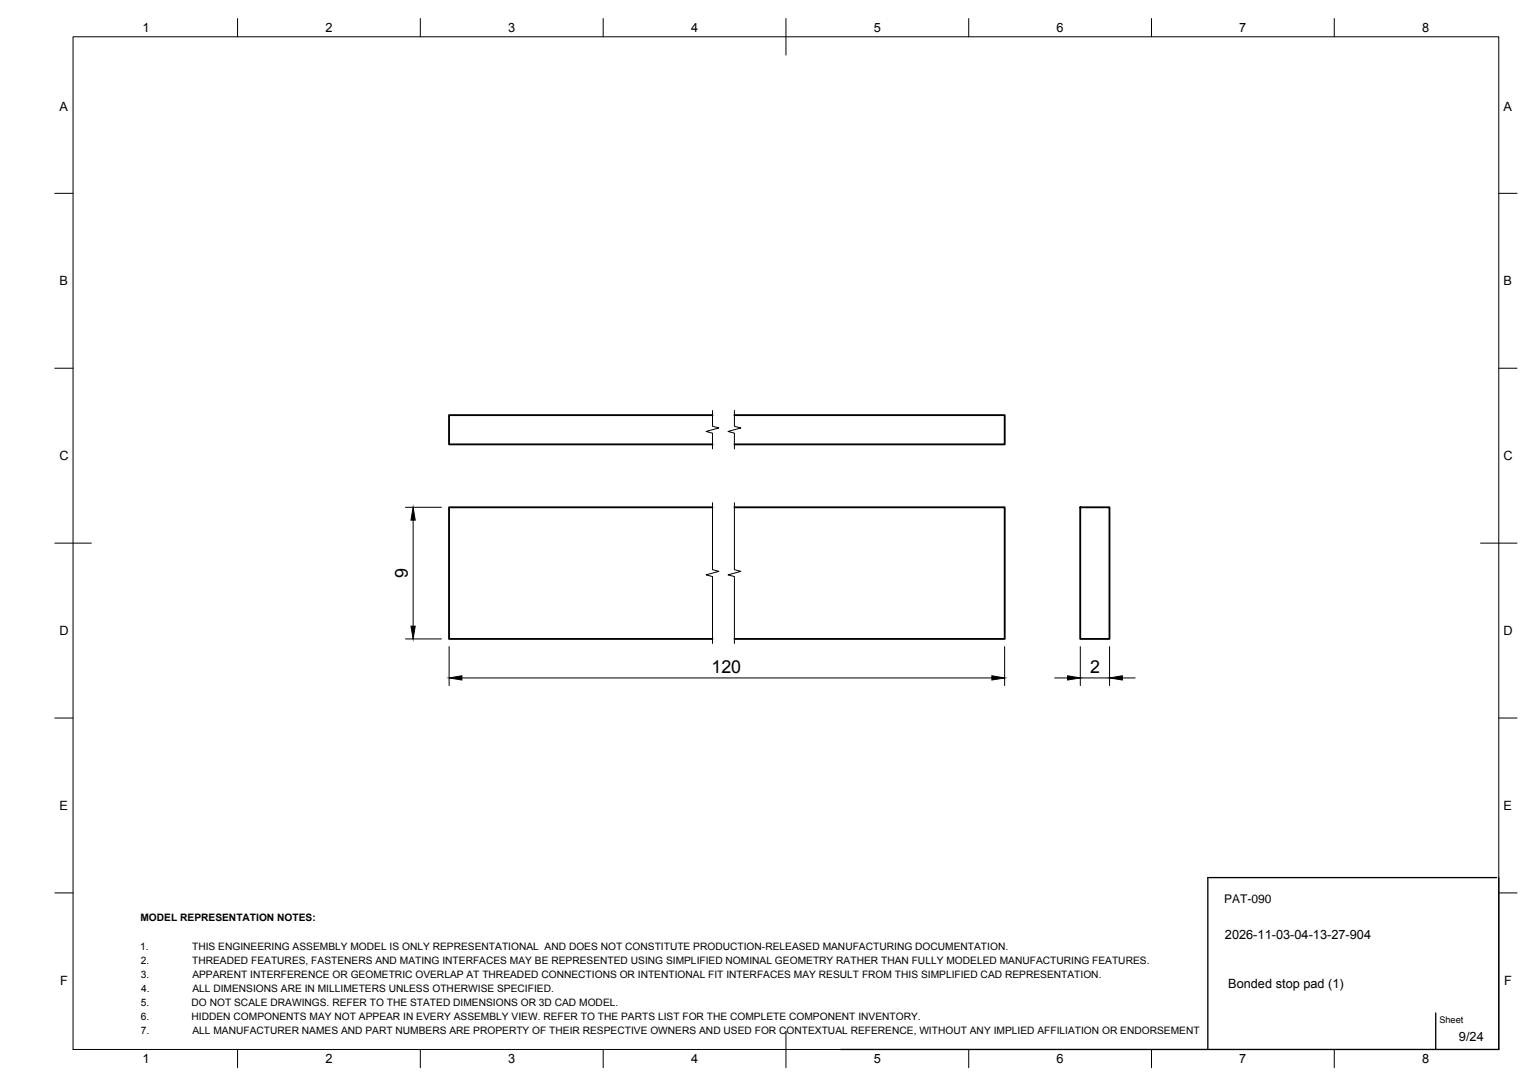
ISO-10303-21;
HEADER;
/* Generated by software containing ST-Developer
 * from STEP Tools, Inc. (www.steptools.com) 
 */

FILE_DESCRIPTION(
/* description */ ('Round-Shaft Linear Stage with Ball Bushings'),
/* implementation_level */ '2;1');

FILE_NAME(
/* name */ 'Bonded stop pad (1).step',
/* time_stamp */ '2026-10-27T10:47:55-07:00',
/* author */ (''),
/* organization */ (''),
/* preprocessor_version */ 'ST-DEVELOPER v20.2',
/* originating_system */ 'Autodesk Translation Framework v15.17.0.0',
/* authorisation */ '');

FILE_SCHEMA (('AUTOMOTIVE_DESIGN { 1 0 10303 214 3 1 1 }'));
ENDSEC;

DATA;
#10=MECHANICAL_DESIGN_GEOMETRIC_PRESENTATION_REPRESENTATION('',(#306),#7835);
#264=SHAPE_REPRESENTATION_RELATIONSHIP('SRR','None',#7952,#285);
#285=ADVANCED_BREP_SHAPE_REPRESENTATION('',(#327),#7816);
#306=STYLED_ITEM('',(#8158),#327);
#327=MANIFOLD_SOLID_BREP('Body1',#4396);
#487=PLANE('',#4744);
#488=PLANE('',#4745);
#489=PLANE('',#4746);
#490=PLANE('',#4747);
#491=PLANE('',#4748);
#492=PLANE('',#4749);
#664=FACE_OUTER_BOUND('',#957,.T.);
#665=FACE_OUTER_BOUND('',#958,.T.);
#666=FACE_OUTER_BOUND('',#959,.T.);
#667=FACE_OUTER_BOUND('',#960,.T.);
#668=FACE_OUTER_BOUND('',#961,.T.);
#669=FACE_OUTER_BOUND('',#962,.T.);
#957=EDGE_LOOP('',(#3210,#3211,#3212,#3213));
#958=EDGE_LOOP('',(#3214,#3215,#3216,#3217));
#959=EDGE_LOOP('',(#3218,#3219,#3220,#3221));
#960=EDGE_LOOP('',(#3222,#3223,#3224,#3225));
#961=EDGE_LOOP('',(#3226,#3227,#3228,#3229));
#962=EDGE_LOOP('',(#3230,#3231,#3232,#3233));
#1317=LINE('',#6808,#1657);
#1318=LINE('',#6810,#1658);
#1319=LINE('',#6812,#1659);
#1320=LINE('',#6813,#1660);
#1321=LINE('',#6816,#1661);
#1322=LINE('',#6818,#1662);
#1323=LINE('',#6819,#1663);
#1324=LINE('',#6822,#1664);
#1325=LINE('',#6824,#1665);
#1326=LINE('',#6825,#1666);
#1327=LINE('',#6827,#1667);
#1328=LINE('',#6828,#1668);
#1657=VECTOR('',#5436,1.);
#1658=VECTOR('',#5437,1.);
#1659=VECTOR('',#5438,1.);
#1660=VECTOR('',#5439,1.);
#1661=VECTOR('',#5442,1.);
#1662=VECTOR('',#5443,1.);
#1663=VECTOR('',#5444,1.);
#1664=VECTOR('',#5447,1.);
#1665=VECTOR('',#5448,1.);
#1666=VECTOR('',#5449,1.);
#1667=VECTOR('',#5452,1.);
#1668=VECTOR('',#5453,1.);
#2190=VERTEX_POINT('',#6806);
#2191=VERTEX_POINT('',#6807);
#2192=VERTEX_POINT('',#6809);
#2193=VERTEX_POINT('',#6811);
#2194=VERTEX_POINT('',#6815);
#2195=VERTEX_POINT('',#6817);
#2196=VERTEX_POINT('',#6821);
#2197=VERTEX_POINT('',#6823);
#2573=EDGE_CURVE('',#2190,#2191,#1317,.T.);
#2574=EDGE_CURVE('',#2191,#2192,#1318,.T.);
#2575=EDGE_CURVE('',#2193,#2192,#1319,.T.);
#2576=EDGE_CURVE('',#2190,#2193,#1320,.T.);
#2577=EDGE_CURVE('',#2194,#2190,#1321,.T.);
#2578=EDGE_CURVE('',#2195,#2193,#1322,.T.);
#2579=EDGE_CURVE('',#2194,#2195,#1323,.T.);
#2580=EDGE_CURVE('',#2196,#2194,#1324,.T.);
#2581=EDGE_CURVE('',#2197,#2195,#1325,.T.);
#2582=EDGE_CURVE('',#2196,#2197,#1326,.T.);
#2583=EDGE_CURVE('',#2191,#2196,#1327,.T.);
#2584=EDGE_CURVE('',#2192,#2197,#1328,.T.);
#3210=ORIENTED_EDGE('',*,*,#2573,.T.);
#3211=ORIENTED_EDGE('',*,*,#2574,.T.);
#3212=ORIENTED_EDGE('',*,*,#2575,.F.);
#3213=ORIENTED_EDGE('',*,*,#2576,.F.);
#3214=ORIENTED_EDGE('',*,*,#2577,.T.);
#3215=ORIENTED_EDGE('',*,*,#2576,.T.);
#3216=ORIENTED_EDGE('',*,*,#2578,.F.);
#3217=ORIENTED_EDGE('',*,*,#2579,.F.);
#3218=ORIENTED_EDGE('',*,*,#2580,.T.);
#3219=ORIENTED_EDGE('',*,*,#2579,.T.);
#3220=ORIENTED_EDGE('',*,*,#2581,.F.);
#3221=ORIENTED_EDGE('',*,*,#2582,.F.);
#3222=ORIENTED_EDGE('',*,*,#2583,.T.);
#3223=ORIENTED_EDGE('',*,*,#2582,.T.);
#3224=ORIENTED_EDGE('',*,*,#2584,.F.);
#3225=ORIENTED_EDGE('',*,*,#2574,.F.);
#3226=ORIENTED_EDGE('',*,*,#2584,.T.);
#3227=ORIENTED_EDGE('',*,*,#2581,.T.);
#3228=ORIENTED_EDGE('',*,*,#2578,.T.);
#3229=ORIENTED_EDGE('',*,*,#2575,.T.);
#3230=ORIENTED_EDGE('',*,*,#2583,.F.);
#3231=ORIENTED_EDGE('',*,*,#2573,.F.);
#3232=ORIENTED_EDGE('',*,*,#2577,.F.);
#3233=ORIENTED_EDGE('',*,*,#2580,.F.);
#4183=ADVANCED_FACE('',(#664),#487,.T.);
#4184=ADVANCED_FACE('',(#665),#488,.T.);
#4185=ADVANCED_FACE('',(#666),#489,.T.);
#4186=ADVANCED_FACE('',(#667),#490,.T.);
#4187=ADVANCED_FACE('',(#668),#491,.T.);
#4188=ADVANCED_FACE('',(#669),#492,.F.);
#4396=CLOSED_SHELL('',(#4183,#4184,#4185,#4186,#4187,#4188));
#4743=AXIS2_PLACEMENT_3D('',#6804,#5432,#5433);
#4744=AXIS2_PLACEMENT_3D('',#6805,#5434,#5435);
#4745=AXIS2_PLACEMENT_3D('',#6814,#5440,#5441);
#4746=AXIS2_PLACEMENT_3D('',#6820,#5445,#5446);
#4747=AXIS2_PLACEMENT_3D('',#6826,#5450,#5451);
#4748=AXIS2_PLACEMENT_3D('',#6829,#5454,#5455);
#4749=AXIS2_PLACEMENT_3D('',#6830,#5456,#5457);
#5432=DIRECTION('axis',(0.,0.,1.));
#5433=DIRECTION('refdir',(1.,0.,0.));
#5434=DIRECTION('center_axis',(0.,1.,0.));
#5435=DIRECTION('ref_axis',(-1.,0.,0.));
#5436=DIRECTION('',(-1.,0.,0.));
#5437=DIRECTION('',(0.,0.,1.));
#5438=DIRECTION('',(-1.,0.,0.));
#5439=DIRECTION('',(0.,0.,1.));
#5440=DIRECTION('center_axis',(1.,0.,0.));
#5441=DIRECTION('ref_axis',(0.,1.,0.));
#5442=DIRECTION('',(0.,1.,0.));
#5443=DIRECTION('',(0.,1.,0.));
#5444=DIRECTION('',(0.,0.,1.));
#5445=DIRECTION('center_axis',(0.,-1.,0.));
#5446=DIRECTION('ref_axis',(1.,0.,0.));
#5447=DIRECTION('',(1.,0.,0.));
#5448=DIRECTION('',(1.,0.,0.));
#5449=DIRECTION('',(0.,0.,1.));
#5450=DIRECTION('center_axis',(-1.,0.,0.));
#5451=DIRECTION('ref_axis',(0.,-1.,0.));
#5452=DIRECTION('',(0.,-1.,0.));
#5453=DIRECTION('',(0.,-1.,0.));
#5454=DIRECTION('center_axis',(0.,0.,1.));
#5455=DIRECTION('ref_axis',(1.,0.,0.));
#5456=DIRECTION('center_axis',(0.,0.,1.));
#5457=DIRECTION('ref_axis',(1.,0.,0.));
#6804=CARTESIAN_POINT('',(0.,0.,0.));
#6805=CARTESIAN_POINT('Origin',(26.,6.,1.6));
#6806=CARTESIAN_POINT('',(26.,6.,1.6));
#6807=CARTESIAN_POINT('',(25.8,6.,1.6));
#6808=CARTESIAN_POINT('',(26.,6.,1.6));
#6809=CARTESIAN_POINT('',(25.8,6.,2.5));
#6810=CARTESIAN_POINT('',(25.8,6.,1.6));
#6811=CARTESIAN_POINT('',(26.,6.,2.5));
#6812=CARTESIAN_POINT('',(26.,6.,2.5));
#6813=CARTESIAN_POINT('',(26.,6.,1.6));
#6814=CARTESIAN_POINT('Origin',(26.,-6.,1.6));
#6815=CARTESIAN_POINT('',(26.,-6.,1.6));
#6816=CARTESIAN_POINT('',(26.,-6.,1.6));
#6817=CARTESIAN_POINT('',(26.,-6.,2.5));
#6818=CARTESIAN_POINT('',(26.,-6.,2.5));
#6819=CARTESIAN_POINT('',(26.,-6.,1.6));
#6820=CARTESIAN_POINT('Origin',(25.8,-6.,1.6));
#6821=CARTESIAN_POINT('',(25.8,-6.,1.6));
#6822=CARTESIAN_POINT('',(25.8,-6.,1.6));
#6823=CARTESIAN_POINT('',(25.8,-6.,2.5));
#6824=CARTESIAN_POINT('',(25.8,-6.,2.5));
#6825=CARTESIAN_POINT('',(25.8,-6.,1.6));
#6826=CARTESIAN_POINT('Origin',(25.8,6.,1.6));
#6827=CARTESIAN_POINT('',(25.8,6.,1.6));
#6828=CARTESIAN_POINT('',(25.8,6.,2.5));
#6829=CARTESIAN_POINT('Origin',(25.9,0.,2.5));
#6830=CARTESIAN_POINT('Origin',(25.9,0.,1.6));
#7790=UNCERTAINTY_MEASURE_WITH_UNIT(LENGTH_MEASURE(0.001),#7836,
'DISTANCE_ACCURACY_VALUE',
'Maximum model space distance between geometric entities at asserted c
onnectivities');
#7809=UNCERTAINTY_MEASURE_WITH_UNIT(LENGTH_MEASURE(0.001),#7836,
'DISTANCE_ACCURACY_VALUE',
'Maximum model space distance between geometric entities at asserted c
onnectivities');
#7816=(
GEOMETRIC_REPRESENTATION_CONTEXT(3)
GLOBAL_UNCERTAINTY_ASSIGNED_CONTEXT((#7790))
GLOBAL_UNIT_ASSIGNED_CONTEXT((#7836,#7838,#7839))
REPRESENTATION_CONTEXT('','3D')
);
#7835=(
GEOMETRIC_REPRESENTATION_CONTEXT(3)
GLOBAL_UNCERTAINTY_ASSIGNED_CONTEXT((#7809))
GLOBAL_UNIT_ASSIGNED_CONTEXT((#7836,#7838,#7839))
REPRESENTATION_CONTEXT('','3D')
);
#7836=(
LENGTH_UNIT()
NAMED_UNIT(*)
SI_UNIT(.CENTI.,.METRE.)
);
#7838=(
NAMED_UNIT(*)
PLANE_ANGLE_UNIT()
SI_UNIT($,.RADIAN.)
);
#7839=(
NAMED_UNIT(*)
SI_UNIT($,.STERADIAN.)
SOLID_ANGLE_UNIT()
);
#7846=SHAPE_DEFINITION_REPRESENTATION(#7871,#7952);
#7871=PRODUCT_DEFINITION_SHAPE('',$,#7978);
#7952=SHAPE_REPRESENTATION('',(#4743),#7816);
#7971=PRODUCT_DEFINITION_CONTEXT('part definition',#8048,'design');
#7978=PRODUCT_DEFINITION('Bonded stop pad (1)','Bonded stop pad (1)',#8003,
#7971);
#8003=PRODUCT_DEFINITION_FORMATION('',$,#8056);
#8048=APPLICATION_CONTEXT(
'Core Data for Automotive Mechanical Design Process');
#8049=PRODUCT_CONTEXT('part definition',#8048,'mechanical');
#8056=PRODUCT('Bonded stop pad (1)','Bonded stop pad (1)',
'Bonded stop pad (1)',(#8049));
#8152=COLOUR_RGB('Off White',0.89,0.88,0.83);
#8153=FILL_AREA_STYLE_COLOUR('',#8152);
#8154=FILL_AREA_STYLE('',(#8153));
#8155=SURFACE_STYLE_FILL_AREA(#8154);
#8156=SURFACE_SIDE_STYLE('',(#8155));
#8157=SURFACE_STYLE_USAGE(.BOTH.,#8156);
#8158=PRESENTATION_STYLE_ASSIGNMENT((#8157));
ENDSEC;
END-ISO-10303-21;
